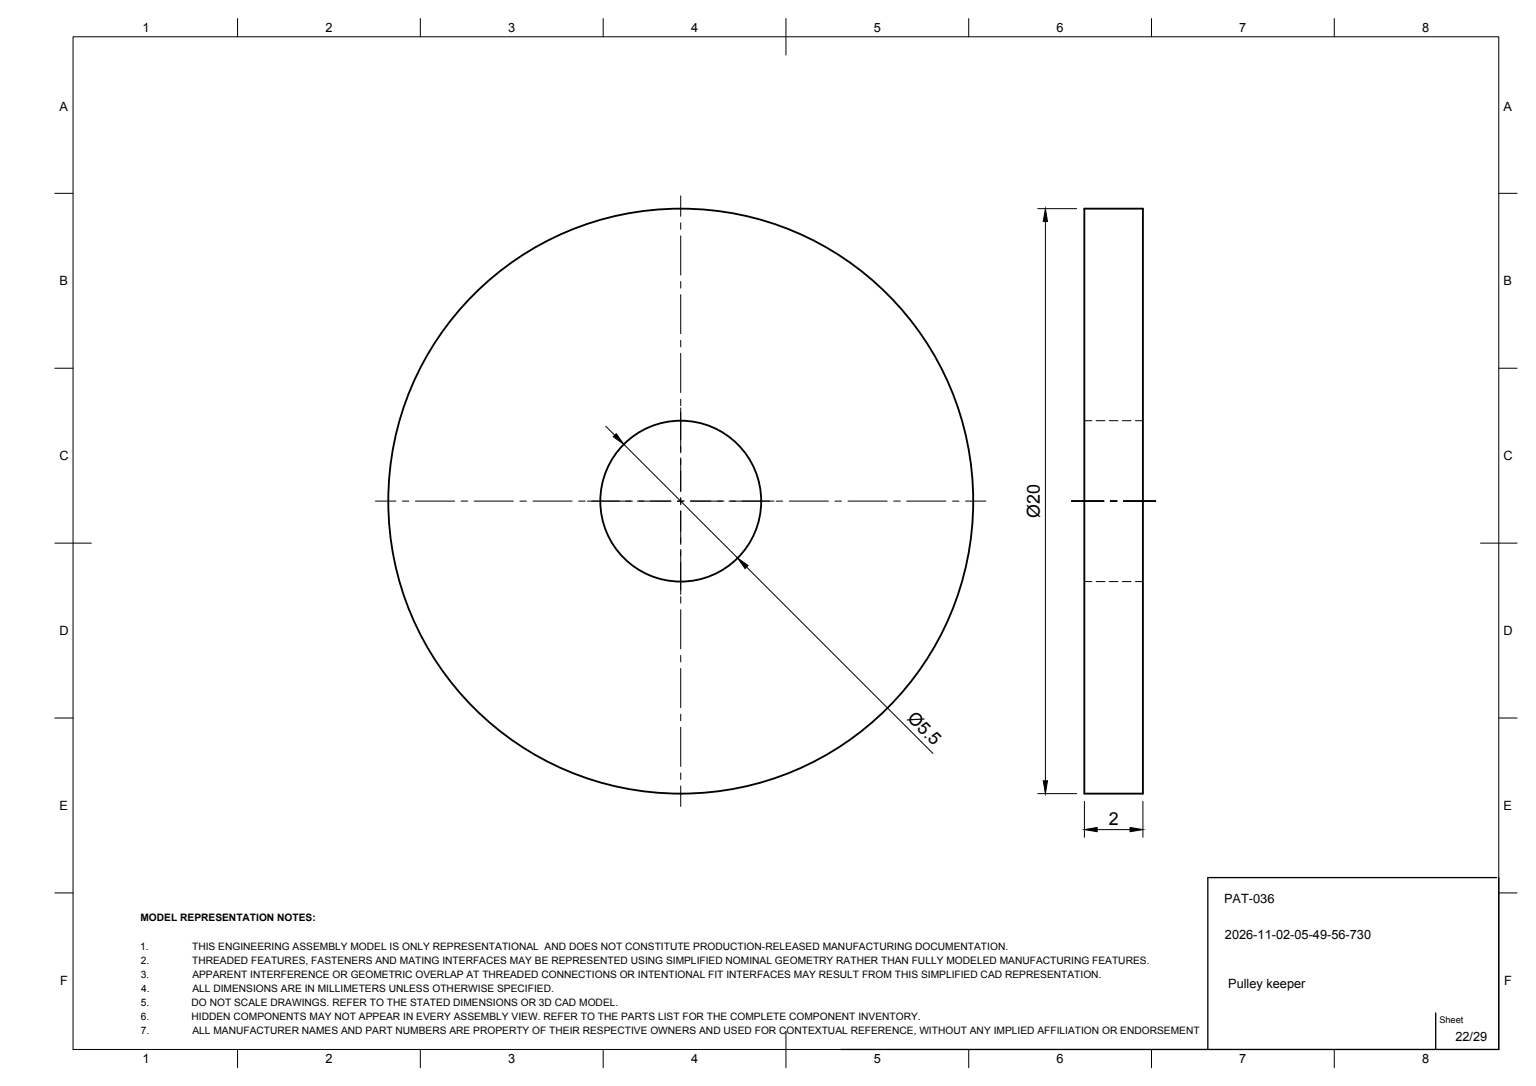
ISO-10303-21;
HEADER;
/* Generated by software containing ST-Developer
 * from STEP Tools, Inc. (www.steptools.com) 
 */

FILE_DESCRIPTION(
/* description */ ('Flange-mounted spindle'),
/* implementation_level */ '2;1');

FILE_NAME(
/* name */ 'Pulley keeper.step',
/* time_stamp */ '2026-10-27T10:49:51-07:00',
/* author */ (''),
/* organization */ (''),
/* preprocessor_version */ 'ST-DEVELOPER v20.2',
/* originating_system */ 'Autodesk Translation Framework v15.17.0.0',
/* authorisation */ '');

FILE_SCHEMA (('AUTOMOTIVE_DESIGN { 1 0 10303 214 3 1 1 }'));
ENDSEC;

DATA;
#10=MECHANICAL_DESIGN_GEOMETRIC_PRESENTATION_REPRESENTATION('',(#354),#11764);
#299=SHAPE_REPRESENTATION_RELATIONSHIP('SRR','None',#11897,#326);
#326=ADVANCED_BREP_SHAPE_REPRESENTATION('',(#380),#11752);
#354=STYLED_ITEM('',(#12113),#380);
#380=MANIFOLD_SOLID_BREP('Body1',#6148);
#461=FACE_BOUND('',#1240,.T.);
#462=FACE_BOUND('',#1242,.T.);
#598=PLANE('',#6732);
#599=PLANE('',#6733);
#822=FACE_OUTER_BOUND('',#1237,.T.);
#823=FACE_OUTER_BOUND('',#1238,.T.);
#824=FACE_OUTER_BOUND('',#1239,.T.);
#825=FACE_OUTER_BOUND('',#1241,.T.);
#1237=EDGE_LOOP('',(#4623,#4624,#4625,#4626));
#1238=EDGE_LOOP('',(#4627,#4628,#4629,#4630));
#1239=EDGE_LOOP('',(#4631));
#1240=EDGE_LOOP('',(#4632));
#1241=EDGE_LOOP('',(#4633));
#1242=EDGE_LOOP('',(#4634));
#1667=LINE('',#10230,#2089);
#1668=LINE('',#10236,#2090);
#2089=VECTOR('',#7934,0.275);
#2090=VECTOR('',#7941,1.);
#2420=CIRCLE('',#6727,0.275);
#2421=CIRCLE('',#6728,0.275);
#2422=CIRCLE('',#6730,1.);
#2423=CIRCLE('',#6731,1.);
#2860=VERTEX_POINT('',#10227);
#2861=VERTEX_POINT('',#10229);
#2862=VERTEX_POINT('',#10233);
#2863=VERTEX_POINT('',#10235);
#3504=EDGE_CURVE('',#2860,#2860,#2420,.T.);
#3505=EDGE_CURVE('',#2860,#2861,#1667,.T.);
#3506=EDGE_CURVE('',#2861,#2861,#2421,.T.);
#3507=EDGE_CURVE('',#2862,#2862,#2422,.T.);
#3508=EDGE_CURVE('',#2862,#2863,#1668,.T.);
#3509=EDGE_CURVE('',#2863,#2863,#2423,.T.);
#4623=ORIENTED_EDGE('',*,*,#3504,.F.);
#4624=ORIENTED_EDGE('',*,*,#3505,.T.);
#4625=ORIENTED_EDGE('',*,*,#3506,.T.);
#4626=ORIENTED_EDGE('',*,*,#3505,.F.);
#4627=ORIENTED_EDGE('',*,*,#3507,.F.);
#4628=ORIENTED_EDGE('',*,*,#3508,.T.);
#4629=ORIENTED_EDGE('',*,*,#3509,.T.);
#4630=ORIENTED_EDGE('',*,*,#3508,.F.);
#4631=ORIENTED_EDGE('',*,*,#3507,.T.);
#4632=ORIENTED_EDGE('',*,*,#3504,.T.);
#4633=ORIENTED_EDGE('',*,*,#3509,.F.);
#4634=ORIENTED_EDGE('',*,*,#3506,.F.);
#5672=CYLINDRICAL_SURFACE('',#6726,0.275);
#5673=CYLINDRICAL_SURFACE('',#6729,1.);
#5933=ADVANCED_FACE('',(#822),#5672,.F.);
#5934=ADVANCED_FACE('',(#823),#5673,.T.);
#5935=ADVANCED_FACE('',(#824,#461),#598,.T.);
#5936=ADVANCED_FACE('',(#825,#462),#599,.F.);
#6148=CLOSED_SHELL('',(#5933,#5934,#5935,#5936));
#6725=AXIS2_PLACEMENT_3D('',#10225,#7928,#7929);
#6726=AXIS2_PLACEMENT_3D('',#10226,#7930,#7931);
#6727=AXIS2_PLACEMENT_3D('',#10228,#7932,#7933);
#6728=AXIS2_PLACEMENT_3D('',#10231,#7935,#7936);
#6729=AXIS2_PLACEMENT_3D('',#10232,#7937,#7938);
#6730=AXIS2_PLACEMENT_3D('',#10234,#7939,#7940);
#6731=AXIS2_PLACEMENT_3D('',#10237,#7942,#7943);
#6732=AXIS2_PLACEMENT_3D('',#10238,#7944,#7945);
#6733=AXIS2_PLACEMENT_3D('',#10239,#7946,#7947);
#7928=DIRECTION('axis',(0.,0.,1.));
#7929=DIRECTION('refdir',(1.,0.,0.));
#7930=DIRECTION('center_axis',(0.,1.,0.));
#7931=DIRECTION('ref_axis',(1.,0.,0.));
#7932=DIRECTION('center_axis',(0.,-1.,0.));
#7933=DIRECTION('ref_axis',(1.,0.,0.));
#7934=DIRECTION('',(0.,-1.,0.));
#7935=DIRECTION('center_axis',(0.,-1.,0.));
#7936=DIRECTION('ref_axis',(1.,0.,0.));
#7937=DIRECTION('center_axis',(0.,1.,0.));
#7938=DIRECTION('ref_axis',(1.,0.,0.));
#7939=DIRECTION('center_axis',(0.,1.,0.));
#7940=DIRECTION('ref_axis',(1.,0.,0.));
#7941=DIRECTION('',(0.,-1.,0.));
#7942=DIRECTION('center_axis',(0.,1.,0.));
#7943=DIRECTION('ref_axis',(1.,0.,0.));
#7944=DIRECTION('center_axis',(0.,1.,0.));
#7945=DIRECTION('ref_axis',(1.,0.,0.));
#7946=DIRECTION('center_axis',(0.,1.,0.));
#7947=DIRECTION('ref_axis',(1.,0.,0.));
#10225=CARTESIAN_POINT('',(0.,0.,0.));
#10226=CARTESIAN_POINT('Origin',(0.,-7.2,8.));
#10227=CARTESIAN_POINT('',(-0.275,-7.,8.));
#10228=CARTESIAN_POINT('Origin',(0.,-7.,8.));
#10229=CARTESIAN_POINT('',(-0.275,-7.2,8.));
#10230=CARTESIAN_POINT('',(-0.275,-7.2,8.));
#10231=CARTESIAN_POINT('Origin',(0.,-7.2,8.));
#10232=CARTESIAN_POINT('Origin',(0.,-7.2,8.));
#10233=CARTESIAN_POINT('',(-1.,-7.,8.));
#10234=CARTESIAN_POINT('Origin',(0.,-7.,8.));
#10235=CARTESIAN_POINT('',(-1.,-7.2,8.));
#10236=CARTESIAN_POINT('',(-1.,-7.2,8.));
#10237=CARTESIAN_POINT('Origin',(0.,-7.2,8.));
#10238=CARTESIAN_POINT('Origin',(0.,-7.,8.));
#10239=CARTESIAN_POINT('Origin',(0.,-7.2,8.));
#11720=UNCERTAINTY_MEASURE_WITH_UNIT(LENGTH_MEASURE(0.001),#11765,
'DISTANCE_ACCURACY_VALUE',
'Maximum model space distance between geometric entities at asserted c
onnectivities');
#11732=UNCERTAINTY_MEASURE_WITH_UNIT(LENGTH_MEASURE(0.001),#11765,
'DISTANCE_ACCURACY_VALUE',
'Maximum model space distance between geometric entities at asserted c
onnectivities');
#11752=(
GEOMETRIC_REPRESENTATION_CONTEXT(3)
GLOBAL_UNCERTAINTY_ASSIGNED_CONTEXT((#11720))
GLOBAL_UNIT_ASSIGNED_CONTEXT((#11765,#11767,#11768))
REPRESENTATION_CONTEXT('','3D')
);
#11764=(
GEOMETRIC_REPRESENTATION_CONTEXT(3)
GLOBAL_UNCERTAINTY_ASSIGNED_CONTEXT((#11732))
GLOBAL_UNIT_ASSIGNED_CONTEXT((#11765,#11767,#11768))
REPRESENTATION_CONTEXT('','3D')
);
#11765=(
LENGTH_UNIT()
NAMED_UNIT(*)
SI_UNIT(.CENTI.,.METRE.)
);
#11767=(
NAMED_UNIT(*)
PLANE_ANGLE_UNIT()
SI_UNIT($,.RADIAN.)
);
#11768=(
NAMED_UNIT(*)
SI_UNIT($,.STERADIAN.)
SOLID_ANGLE_UNIT()
);
#11788=SHAPE_DEFINITION_REPRESENTATION(#11821,#11897);
#11821=PRODUCT_DEFINITION_SHAPE('',$,#11929);
#11897=SHAPE_REPRESENTATION('',(#6725),#11752);
#11909=PRODUCT_DEFINITION_CONTEXT('part definition',#12004,'design');
#11929=PRODUCT_DEFINITION('Pulley keeper','Pulley keeper',#11960,#11909);
#11960=PRODUCT_DEFINITION_FORMATION('',$,#12025);
#12004=APPLICATION_CONTEXT(
'Core Data for Automotive Mechanical Design Process');
#12005=PRODUCT_CONTEXT('part definition',#12004,'mechanical');
#12025=PRODUCT('Pulley keeper','Pulley keeper','Pulley keeper',(#12005));
#12107=COLOUR_RGB('Off White',0.89,0.88,0.83);
#12108=FILL_AREA_STYLE_COLOUR('',#12107);
#12109=FILL_AREA_STYLE('',(#12108));
#12110=SURFACE_STYLE_FILL_AREA(#12109);
#12111=SURFACE_SIDE_STYLE('',(#12110));
#12112=SURFACE_STYLE_USAGE(.BOTH.,#12111);
#12113=PRESENTATION_STYLE_ASSIGNMENT((#12112));
ENDSEC;
END-ISO-10303-21;
